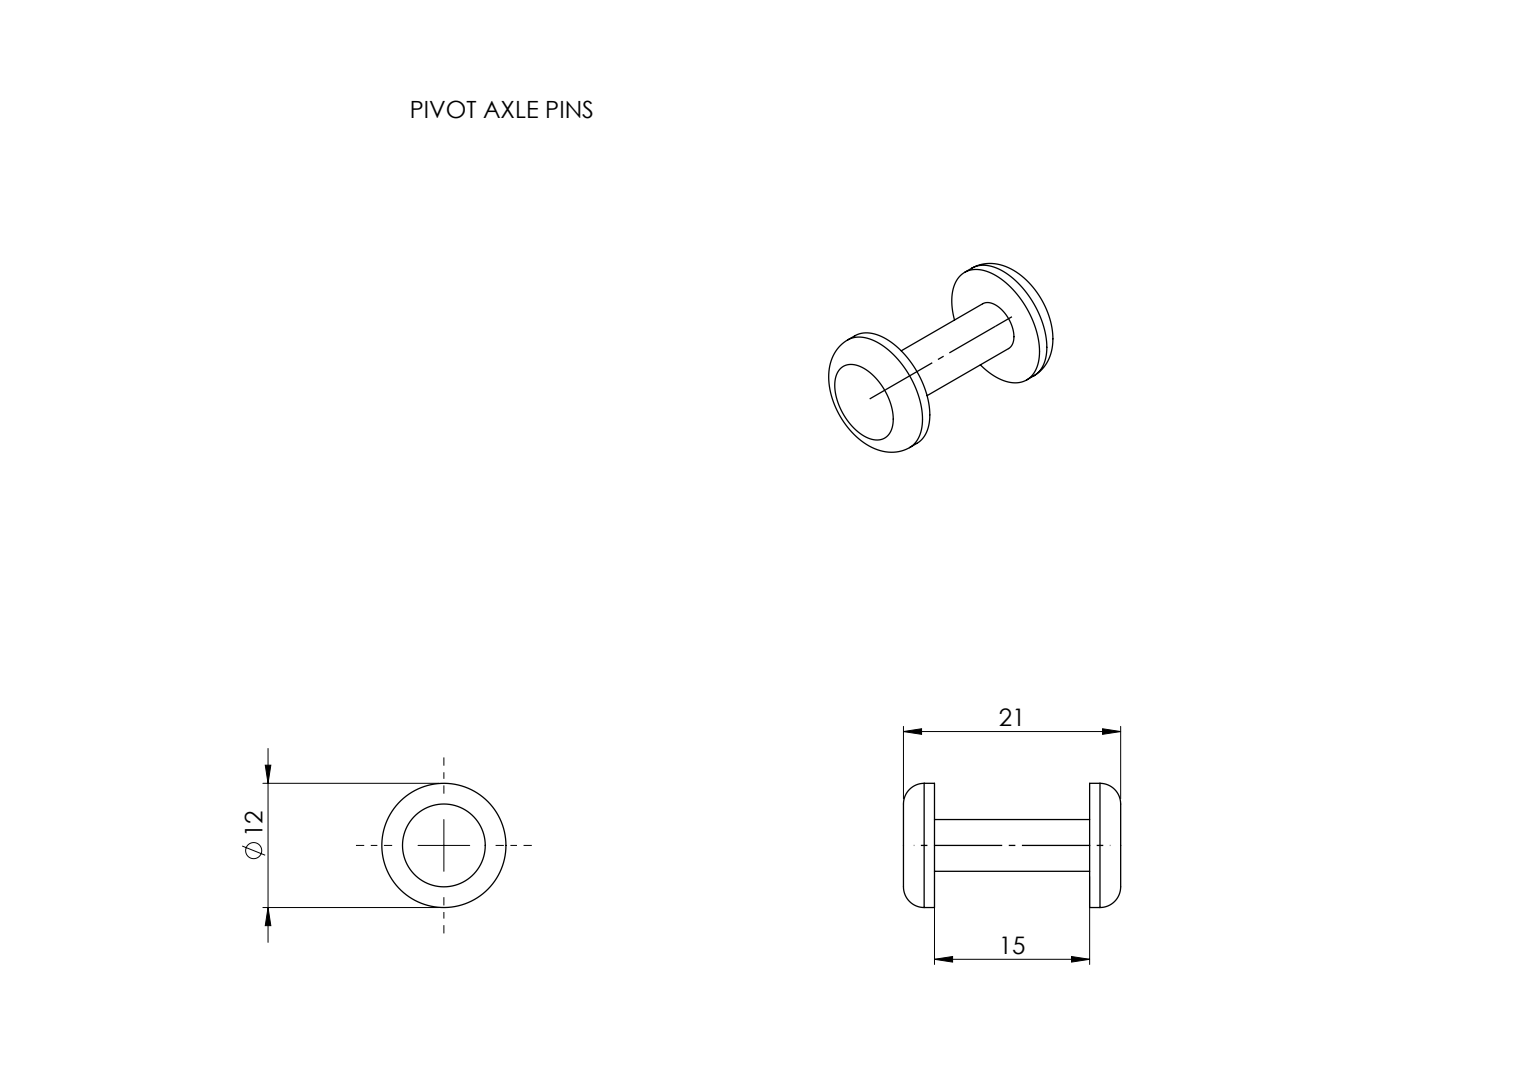
ISO-10303-21;
HEADER;
FILE_DESCRIPTION (('STEP AP214'),
    '1' );
FILE_NAME ('Pivot Axle Pins.step',
    '2026-10-08T14:03:35',
    ( '' ),
    ( '' ),
    'SwSTEP 2.0',
    'SolidWorks 2026',
    '' );
FILE_SCHEMA (( 'AUTOMOTIVE_DESIGN' ));
ENDSEC;

DATA;
#5=CIRCLE ( 'NONE', #8996, 5.999999999999998224 ) ;
#23=AXIS2_PLACEMENT_3D ( 'NONE', #10959, #4438, #5501 ) ;
#42=VERTEX_POINT ( 'NONE', #3602 ) ;
#77=FACE_BOUND ( 'NONE', #7085, .T. ) ;
#131=VERTEX_POINT ( 'NONE', #11545 ) ;
#137=AXIS2_PLACEMENT_3D ( 'NONE', #11805, #13167, #2478 ) ;
#178=DIRECTION ( 'NONE',  ( 1.000000000000000000, 0.000000000000000000, 0.000000000000000000 ) ) ;
#205=PLANE ( 'NONE',  #6332 ) ;
#210=ORIENTED_EDGE ( 'NONE', *, *, #10551, .T. ) ;
#257=DIRECTION ( 'NONE',  ( -0.000000000000000000, -0.000000000000000000, 1.000000000000000000 ) ) ;
#382=DIRECTION ( 'NONE',  ( 1.000000000000000000, 0.000000000000000000, 0.000000000000000000 ) ) ;
#411=FILL_AREA_STYLE_COLOUR ( '', #8311 ) ;
#418=ORIENTED_EDGE ( 'NONE', *, *, #4130, .F. ) ;
#427=EDGE_LOOP ( 'NONE', ( #12636, #418, #9896, #533 ) ) ;
#447=PLANE ( 'NONE',  #3696 ) ;
#454=AXIS2_PLACEMENT_3D ( 'NONE', #3228, #2248, #4282 ) ;
#492=PRODUCT_CONTEXT ( 'NONE', #10764, 'mechanical' ) ;
#533=ORIENTED_EDGE ( 'NONE', *, *, #2253, .T. ) ;
#560=EDGE_CURVE ( 'NONE', #8899, #4393, #6700, .T. ) ;
#567=CARTESIAN_POINT ( 'NONE',  ( -35.00000000000000000, -4.286263797015736496E-15, -7.500000000000000000 ) ) ;
#579=CARTESIAN_POINT ( 'NONE',  ( -41.00000000000000000, -4.286263797015736496E-15, 7.500000000000000000 ) ) ;
#591=SURFACE_STYLE_USAGE ( .BOTH. , #5908 ) ;
#768=VERTEX_POINT ( 'NONE', #9967 ) ;
#794=DIRECTION ( 'NONE',  ( 0.000000000000000000, 0.000000000000000000, 1.000000000000000000 ) ) ;
#835=CIRCLE ( 'NONE', #11129, 5.999999999999998224 ) ;
#888=CARTESIAN_POINT ( 'NONE',  ( -41.00000000000000000, -4.286263797015736496E-15, -10.49999999999999822 ) ) ;
#918=CYLINDRICAL_SURFACE ( 'NONE', #6361, 2.500000000000002220 ) ;
#963=LINE ( 'NONE', #2075, #5370 ) ;
#965=DIRECTION ( 'NONE',  ( -0.000000000000000000, -0.000000000000000000, -1.000000000000000000 ) ) ;
#1032=DIRECTION ( 'NONE',  ( -0.000000000000000000, -0.000000000000000000, -1.000000000000000000 ) ) ;
#1033=DIRECTION ( 'NONE',  ( -1.000000000000000000, 0.000000000000000000, 0.000000000000000000 ) ) ;
#1081=DIRECTION ( 'NONE',  ( -0.000000000000000000, -0.000000000000000000, 1.000000000000000000 ) ) ;
#1112=SURFACE_STYLE_USAGE ( .BOTH. , #4254 ) ;
#1158=ORIENTED_EDGE ( 'NONE', *, *, #4130, .T. ) ;
#1226=VERTEX_POINT ( 'NONE', #6896 ) ;
#1235=DIRECTION ( 'NONE',  ( 0.000000000000000000, 0.000000000000000000, -1.000000000000000000 ) ) ;
#1341=CARTESIAN_POINT ( 'NONE',  ( -39.00000000000000000, -4.776122516674677878E-15, -8.499999999999998224 ) ) ;
#1345=CARTESIAN_POINT ( 'NONE',  ( -35.00000000000000000, -4.286263797015736496E-15, -7.500000000000000000 ) ) ;
#1409=CARTESIAN_POINT ( 'NONE',  ( 0.000000000000000000, 0.000000000000000000, 0.000000000000000000 ) ) ;
#1434=CIRCLE ( 'NONE', #6806, 3.999999999999996447 ) ;
#1443=VECTOR ( 'NONE', #13173, 1000.000000000000000 ) ;
#1461=STYLED_ITEM ( 'NONE', ( #12222 ), #5559 ) ;
#1462=EDGE_LOOP ( 'NONE', ( #2845, #13234, #8779, #12885 ) ) ;
#1505=CARTESIAN_POINT ( 'NONE',  ( -35.00000000000000000, -4.286263797015736496E-15, 7.500000000000000000 ) ) ;
#1524=UNCERTAINTY_MEASURE_WITH_UNIT (LENGTH_MEASURE( 1.000000000000000082E-05 ), #2490, 'distance_accuracy_value', 'NONE');
#1595=STYLED_ITEM ( 'NONE', ( #6768 ), #7994 ) ;
#1604=ORIENTED_EDGE ( 'NONE', *, *, #8953, .F. ) ;
#1623=SHAPE_REPRESENTATION_RELATIONSHIP ( 'NONE' , 'NONE' ,  #3787, #5559 ) ;
#1647=CYLINDRICAL_SURFACE ( 'NONE', #7272, 5.999999999999998224 ) ;
#1667=CARTESIAN_POINT ( 'NONE',  ( -35.00000000000000000, -4.286263797015736496E-15, 10.49999999999999822 ) ) ;
#1691=AXIS2_PLACEMENT_3D ( 'NONE', #9348, #794, #9415 ) ;
#1746=CARTESIAN_POINT ( 'NONE',  ( -37.50000000000000711, -4.286263797015736496E-15, 7.500000000000000000 ) ) ;
#1782=CARTESIAN_POINT ( 'NONE',  ( -29.00000000000000355, -3.551475717527324818E-15, 8.499999999999998224 ) ) ;
#1783=DIRECTION ( 'NONE',  ( 0.000000000000000000, 0.000000000000000000, 1.000000000000000000 ) ) ;
#1851=CYLINDRICAL_SURFACE ( 'NONE', #13242, 5.999999999999998224 ) ;
#1939=DIRECTION ( 'NONE',  ( -0.000000000000000000, -0.000000000000000000, 1.000000000000000000 ) ) ;
#1990=VECTOR ( 'NONE', #3207, 1000.000000000000000 ) ;
#2036=CARTESIAN_POINT ( 'NONE',  ( -35.00000000000000000, -4.286263797015736496E-15, 7.500000000000000000 ) ) ;
#2075=CARTESIAN_POINT ( 'NONE',  ( -41.00000000000000000, -4.286263797015736496E-15, 10.49999999999999822 ) ) ;
#2089=LINE ( 'NONE', #5313, #1990 ) ;
#2155=CARTESIAN_POINT ( 'NONE',  ( -35.00000000000000000, -4.286263797015736496E-15, 10.49999999999999822 ) ) ;
#2225=AXIS2_PLACEMENT_3D ( 'NONE', #9848, #257, #4510 ) ;
#2247=EDGE_CURVE ( 'NONE', #4900, #4459, #5, .T. ) ;
#2248=DIRECTION ( 'NONE',  ( -0.000000000000000000, -0.000000000000000000, 1.000000000000000000 ) ) ;
#2253=EDGE_CURVE ( 'NONE', #12007, #13310, #11863, .T. ) ;
#2278=CARTESIAN_POINT ( 'NONE',  ( -35.00000000000000000, -4.286263797015736496E-15, -8.499999999999998224 ) ) ;
#2353=AXIS2_PLACEMENT_3D ( 'NONE', #10131, #5844, #11094 ) ;
#2414=TOROIDAL_SURFACE ( 'NONE', #9155, 3.999999999999998224, 2.000000000000000000 ) ;
#2478=DIRECTION ( 'NONE',  ( 1.000000000000000000, 0.000000000000000000, 0.000000000000000000 ) ) ;
#2490=( LENGTH_UNIT ( ) NAMED_UNIT ( * ) SI_UNIT ( .MILLI., .METRE. ) );
#2497=EDGE_CURVE ( 'NONE', #42, #4459, #963, .T. ) ;
#2580=CIRCLE ( 'NONE', #137, 3.999999999999996447 ) ;
#2658=ORIENTED_EDGE ( 'NONE', *, *, #11315, .T. ) ;
#2672=EDGE_CURVE ( 'NONE', #13647, #8899, #5165, .T. ) ;
#2673=EDGE_CURVE ( 'NONE', #8113, #42, #9191, .T. ) ;
#2756=VECTOR ( 'NONE', #8329, 1000.000000000000000 ) ;
#2766=EDGE_LOOP ( 'NONE', ( #12928, #8220 ) ) ;
#2810=ORIENTED_EDGE ( 'NONE', *, *, #3408, .F. ) ;
#2845=ORIENTED_EDGE ( 'NONE', *, *, #6497, .F. ) ;
#2885=FILL_AREA_STYLE ('',( #4706 ) ) ;
#2895=CIRCLE ( 'NONE', #3105, 2.500000000000002220 ) ;
#2897=EDGE_LOOP ( 'NONE', ( #1158, #7841 ) ) ;
#2955=CARTESIAN_POINT ( 'NONE',  ( -35.00000000000000000, -4.286263797015736496E-15, 7.500000000000000000 ) ) ;
#2983=AXIS2_PLACEMENT_3D ( 'NONE', #3063, #965, #13827 ) ;
#3035=MECHANICAL_DESIGN_GEOMETRIC_PRESENTATION_REPRESENTATION('',(#1461),#6605);
#3063=CARTESIAN_POINT ( 'NONE',  ( -35.00000000000000000, -4.286263797015736496E-15, 8.499999999999998224 ) ) ;
#3105=AXIS2_PLACEMENT_3D ( 'NONE', #567, #7912, #6713 ) ;
#3157=ORIENTED_EDGE ( 'NONE', *, *, #8437, .T. ) ;
#3207=DIRECTION ( 'NONE',  ( -0.000000000000000000, -0.000000000000000000, -1.000000000000000000 ) ) ;
#3227=VECTOR ( 'NONE', #1939, 1000.000000000000000 ) ;
#3228=CARTESIAN_POINT ( 'NONE',  ( -35.00000000000000000, -4.286263797015736496E-15, -10.49999999999999822 ) ) ;
#3286=PLANE ( 'NONE',  #11612 ) ;
#3317=DIRECTION ( 'NONE',  ( -1.000000000000000000, 1.224646799147353454E-16, 0.000000000000000000 ) ) ;
#3345=TOROIDAL_SURFACE ( 'NONE', #6937, 3.999999999999998224, 2.000000000000000000 ) ;
#3364=MECHANICAL_DESIGN_GEOMETRIC_PRESENTATION_REPRESENTATION('',(#1595),#8521);
#3392=CARTESIAN_POINT ( 'NONE',  ( -31.00000000000000711, -4.286263797015736496E-15, 10.49999999999999822 ) ) ;
#3408=EDGE_CURVE ( 'NONE', #8113, #12059, #3837, .T. ) ;
#3482=DIRECTION ( 'NONE',  ( 0.000000000000000000, 0.000000000000000000, -1.000000000000000000 ) ) ;
#3502=DIRECTION ( 'NONE',  ( -1.000000000000000000, 0.000000000000000000, 0.000000000000000000 ) ) ;
#3505=DIRECTION ( 'NONE',  ( 1.000000000000000000, 1.224646799147353454E-16, 0.000000000000000000 ) ) ;
#3513=DIRECTION ( 'NONE',  ( 0.000000000000000000, 0.000000000000000000, 1.000000000000000000 ) ) ;
#3583=EDGE_LOOP ( 'NONE', ( #5772, #5608, #6832, #5918 ) ) ;
#3589=DIRECTION ( 'NONE',  ( 1.000000000000000000, 0.000000000000000000, 0.000000000000000000 ) ) ;
#3602=CARTESIAN_POINT ( 'NONE',  ( -41.00000000000000000, -4.286263797015736496E-15, 8.499999999999998224 ) ) ;
#3628=ADVANCED_FACE ( 'NONE', ( #9017, #13324 ), #7110, .F. ) ;
#3691=SHAPE_DEFINITION_REPRESENTATION ( #13049, #3787 ) ;
#3696=AXIS2_PLACEMENT_3D ( 'NONE', #12146, #6813, #11088 ) ;
#3750=DIRECTION ( 'NONE',  ( 0.000000000000000000, 0.000000000000000000, 1.000000000000000000 ) ) ;
#3787=SHAPE_REPRESENTATION ( 'Pivot Axle Pins', ( #8193 ), #13606 ) ;
#3837=CIRCLE ( 'NONE', #11670, 2.000000000000000000 ) ;
#3913=AXIS2_PLACEMENT_3D ( 'NONE', #5709, #13099, #3317 ) ;
#3937=( LENGTH_UNIT ( ) NAMED_UNIT ( * ) SI_UNIT ( .MILLI., .METRE. ) );
#3954=DIRECTION ( 'NONE',  ( -0.000000000000000000, -0.000000000000000000, -1.000000000000000000 ) ) ;
#3996=AXIS2_PLACEMENT_3D ( 'NONE', #2155, #4392, #9664 ) ;
#4130=EDGE_CURVE ( 'NONE', #4461, #8031, #12976, .T. ) ;
#4136=DIRECTION ( 'NONE',  ( 1.000000000000000000, 0.000000000000000000, 0.000000000000000000 ) ) ;
#4155=PRODUCT_DEFINITION_FORMATION_WITH_SPECIFIED_SOURCE ( 'ANY', '', #9019, .NOT_KNOWN. ) ;
#4254=SURFACE_SIDE_STYLE ('',( #4588 ) ) ;
#4282=DIRECTION ( 'NONE',  ( 1.000000000000000000, 0.000000000000000000, 0.000000000000000000 ) ) ;
#4383=ADVANCED_FACE ( 'NONE', ( #77, #8614 ), #3286, .F. ) ;
#4392=DIRECTION ( 'NONE',  ( -0.000000000000000000, -0.000000000000000000, -1.000000000000000000 ) ) ;
#4393=VERTEX_POINT ( 'NONE', #9811 ) ;
#4438=DIRECTION ( 'NONE',  ( -0.000000000000000000, -0.000000000000000000, -1.000000000000000000 ) ) ;
#4441=CARTESIAN_POINT ( 'NONE',  ( -37.50000000000000711, -4.286263797015736496E-15, -7.500000000000000000 ) ) ;
#4458=ADVANCED_FACE ( 'NONE', ( #10306 ), #2414, .T. ) ;
#4459=VERTEX_POINT ( 'NONE', #579 ) ;
#4461=VERTEX_POINT ( 'NONE', #1746 ) ;
#4510=DIRECTION ( 'NONE',  ( 1.000000000000000000, 0.000000000000000000, 0.000000000000000000 ) ) ;
#4588=SURFACE_STYLE_FILL_AREA ( #12758 ) ;
#4592=CIRCLE ( 'NONE', #2353, 5.999999999999998224 ) ;
#4689=AXIS2_PLACEMENT_3D ( 'NONE', #4801, #8938, #3513 ) ;
#4706=FILL_AREA_STYLE_COLOUR ( '', #10205 ) ;
#4761=DIRECTION ( 'NONE',  ( 1.000000000000000000, 0.000000000000000000, 0.000000000000000000 ) ) ;
#4801=CARTESIAN_POINT ( 'NONE',  ( -31.00000000000000711, -4.286263797015736496E-15, -8.499999999999998224 ) ) ;
#4806=CARTESIAN_POINT ( 'NONE',  ( -41.00000000000000000, -4.286263797015736496E-15, -8.499999999999998224 ) ) ;
#4823=EDGE_CURVE ( 'NONE', #1226, #768, #835, .T. ) ;
#4900=VERTEX_POINT ( 'NONE', #8326 ) ;
#4936=CIRCLE ( 'NONE', #8724, 3.999999999999996447 ) ;
#5071=ORIENTED_EDGE ( 'NONE', *, *, #2672, .F. ) ;
#5076=DIRECTION ( 'NONE',  ( -1.000000000000000000, 0.000000000000000000, 0.000000000000000000 ) ) ;
#5115=ORIENTED_EDGE ( 'NONE', *, *, #5924, .T. ) ;
#5126=FACE_OUTER_BOUND ( 'NONE', #5614, .T. ) ;
#5165=CIRCLE ( 'NONE', #10093, 5.999999999999998224 ) ;
#5175=CARTESIAN_POINT ( 'NONE',  ( -31.00000000000000711, -4.286263797015736496E-15, 8.499999999999998224 ) ) ;
#5191=DIRECTION ( 'NONE',  ( 0.000000000000000000, 0.000000000000000000, 1.000000000000000000 ) ) ;
#5252=ORIENTED_EDGE ( 'NONE', *, *, #13339, .F. ) ;
#5299=DIRECTION ( 'NONE',  ( -0.000000000000000000, -0.000000000000000000, 1.000000000000000000 ) ) ;
#5313=CARTESIAN_POINT ( 'NONE',  ( -29.00000000000000355, -3.551475717527324818E-15, 10.49999999999999822 ) ) ;
#5348=CLOSED_SHELL ( 'NONE', ( #7075, #11998, #12703, #8925, #11450, #10014, #13692, #5636, #3628, #12289, #4383, #7452, #10791, #4458 ) ) ;
#5366=ORIENTED_EDGE ( 'NONE', *, *, #4823, .T. ) ;
#5370=VECTOR ( 'NONE', #1032, 1000.000000000000000 ) ;
#5501=DIRECTION ( 'NONE',  ( 1.000000000000000000, 0.000000000000000000, 0.000000000000000000 ) ) ;
#5549=CARTESIAN_POINT ( 'NONE',  ( -35.00000000000000000, -4.286263797015736496E-15, 7.500000000000000000 ) ) ;
#5556=CARTESIAN_POINT ( 'NONE',  ( -37.50000000000000711, -4.286263797015736496E-15, 7.500000000000000000 ) ) ;
#5559=ADVANCED_BREP_SHAPE_REPRESENTATION ( '', ( #7994, #8193 ), #13606 ) ;
#5581=CIRCLE ( 'NONE', #2225, 5.999999999999998224 ) ;
#5607=VERTEX_POINT ( 'NONE', #13196 ) ;
#5608=ORIENTED_EDGE ( 'NONE', *, *, #2673, .F. ) ;
#5614=EDGE_LOOP ( 'NONE', ( #11627, #210, #7003, #2810 ) ) ;
#5636=ADVANCED_FACE ( 'NONE', ( #7547 ), #205, .T. ) ;
#5639=FACE_OUTER_BOUND ( 'NONE', #10808, .T. ) ;
#5709=CARTESIAN_POINT ( 'NONE',  ( -39.00000000000000000, -3.796405077356795904E-15, 8.499999999999998224 ) ) ;
#5761=FACE_OUTER_BOUND ( 'NONE', #12496, .T. ) ;
#5772=ORIENTED_EDGE ( 'NONE', *, *, #10551, .F. ) ;
#5785=DIRECTION ( 'NONE',  ( 0.000000000000000000, 0.000000000000000000, -1.000000000000000000 ) ) ;
#5800=AXIS2_PLACEMENT_3D ( 'NONE', #10517, #5191, #4136 ) ;
#5825=ORIENTED_EDGE ( 'NONE', *, *, #2497, .T. ) ;
#5842=EDGE_CURVE ( 'NONE', #8031, #13310, #7403, .T. ) ;
#5844=DIRECTION ( 'NONE',  ( 0.000000000000000000, 0.000000000000000000, -1.000000000000000000 ) ) ;
#5882=DIRECTION ( 'NONE',  ( 0.000000000000000000, 0.000000000000000000, 1.000000000000000000 ) ) ;
#5908=SURFACE_SIDE_STYLE ('',( #10249 ) ) ;
#5917=ORIENTED_EDGE ( 'NONE', *, *, #13339, .T. ) ;
#5918=ORIENTED_EDGE ( 'NONE', *, *, #10219, .F. ) ;
#5924=EDGE_CURVE ( 'NONE', #42, #8113, #8346, .T. ) ;
#5968=DIRECTION ( 'NONE',  ( 1.000000000000000000, 0.000000000000000000, 0.000000000000000000 ) ) ;
#6049=( NAMED_UNIT ( * ) SI_UNIT ( $, .STERADIAN. ) SOLID_ANGLE_UNIT ( ) );
#6069=DIRECTION ( 'NONE',  ( 0.000000000000000000, 0.000000000000000000, 1.000000000000000000 ) ) ;
#6091=CARTESIAN_POINT ( 'NONE',  ( -32.50000000000000000, -3.980102097228898626E-15, 7.500000000000000000 ) ) ;
#6131=AXIS2_PLACEMENT_3D ( 'NONE', #2036, #10587, #8480 ) ;
#6194=DIRECTION ( 'NONE',  ( -1.000000000000000000, 0.000000000000000000, 0.000000000000000000 ) ) ;
#6332=AXIS2_PLACEMENT_3D ( 'NONE', #12039, #11764, #7683 ) ;
#6354=CYLINDRICAL_SURFACE ( 'NONE', #12250, 5.999999999999998224 ) ;
#6359=ORIENTED_EDGE ( 'NONE', *, *, #2253, .F. ) ;
#6361=AXIS2_PLACEMENT_3D ( 'NONE', #2955, #7221, #11504 ) ;
#6494=CIRCLE ( 'NONE', #10947, 5.999999999999998224 ) ;
#6497=EDGE_CURVE ( 'NONE', #8031, #4461, #11934, .T. ) ;
#6589=ORIENTED_EDGE ( 'NONE', *, *, #11075, .T. ) ;
#6605=( GEOMETRIC_REPRESENTATION_CONTEXT ( 3 ) GLOBAL_UNCERTAINTY_ASSIGNED_CONTEXT ( ( #13351 ) ) GLOBAL_UNIT_ASSIGNED_CONTEXT ( ( #3937, #8082, #6049 ) ) REPRESENTATION_CONTEXT ( 'NONE', 'WORKASPACE' ) );
#6634=ORIENTED_EDGE ( 'NONE', *, *, #560, .T. ) ;
#6700=CIRCLE ( 'NONE', #4689, 2.000000000000000000 ) ;
#6713=DIRECTION ( 'NONE',  ( 1.000000000000000000, 0.000000000000000000, 0.000000000000000000 ) ) ;
#6723=CARTESIAN_POINT ( 'NONE',  ( -35.00000000000000000, -4.286263797015736496E-15, -7.500000000000000000 ) ) ;
#6754=DIRECTION ( 'NONE',  ( 0.000000000000000000, 0.000000000000000000, 1.000000000000000000 ) ) ;
#6768=PRESENTATION_STYLE_ASSIGNMENT (( #1112 ) ) ;
#6806=AXIS2_PLACEMENT_3D ( 'NONE', #1667, #5882, #10223 ) ;
#6813=DIRECTION ( 'NONE',  ( 0.000000000000000000, 0.000000000000000000, -1.000000000000000000 ) ) ;
#6832=ORIENTED_EDGE ( 'NONE', *, *, #3408, .T. ) ;
#6842=( NAMED_UNIT ( * ) PLANE_ANGLE_UNIT ( ) SI_UNIT ( $, .RADIAN. ) );
#6896=CARTESIAN_POINT ( 'NONE',  ( -41.00000000000000000, -4.286263797015736496E-15, -7.500000000000000000 ) ) ;
#6937=AXIS2_PLACEMENT_3D ( 'NONE', #10958, #9714, #10818 ) ;
#7003=ORIENTED_EDGE ( 'NONE', *, *, #7538, .F. ) ;
#7010=APPLICATION_CONTEXT ( 'automotive_design' ) ;
#7044=CIRCLE ( 'NONE', #3913, 2.000000000000001776 ) ;
#7075=ADVANCED_FACE ( 'NONE', ( #5639 ), #3345, .T. ) ;
#7085=EDGE_LOOP ( 'NONE', ( #6359, #1604 ) ) ;
#7110=PLANE ( 'NONE',  #8756 ) ;
#7140=EDGE_CURVE ( 'NONE', #768, #1226, #5581, .T. ) ;
#7151=EDGE_CURVE ( 'NONE', #4459, #4900, #6494, .T. ) ;
#7160=CARTESIAN_POINT ( 'NONE',  ( -35.00000000000000000, -4.286263797015736496E-15, 7.500000000000000000 ) ) ;
#7179=FACE_OUTER_BOUND ( 'NONE', #10615, .T. ) ;
#7221=DIRECTION ( 'NONE',  ( -0.000000000000000000, -0.000000000000000000, -1.000000000000000000 ) ) ;
#7272=AXIS2_PLACEMENT_3D ( 'NONE', #13601, #3954, #5076 ) ;
#7317=FACE_OUTER_BOUND ( 'NONE', #3583, .T. ) ;
#7403=LINE ( 'NONE', #6091, #2756 ) ;
#7452=ADVANCED_FACE ( 'NONE', ( #7179 ), #1851, .T. ) ;
#7485=CYLINDRICAL_SURFACE ( 'NONE', #3996, 5.999999999999998224 ) ;
#7538=EDGE_CURVE ( 'NONE', #12059, #131, #4936, .T. ) ;
#7547=FACE_OUTER_BOUND ( 'NONE', #13469, .T. ) ;
#7569=ORIENTED_EDGE ( 'NONE', *, *, #8901, .F. ) ;
#7683=DIRECTION ( 'NONE',  ( 1.000000000000000000, 0.000000000000000000, -0.000000000000000000 ) ) ;
#7790=ORIENTED_EDGE ( 'NONE', *, *, #7151, .T. ) ;
#7841=ORIENTED_EDGE ( 'NONE', *, *, #6497, .T. ) ;
#7912=DIRECTION ( 'NONE',  ( 0.000000000000000000, 0.000000000000000000, 1.000000000000000000 ) ) ;
#7962=DIRECTION ( 'NONE',  ( 1.000000000000000000, 0.000000000000000000, 0.000000000000000000 ) ) ;
#7994=MANIFOLD_SOLID_BREP ( 'Mirror3', #5348 ) ;
#7996=CARTESIAN_POINT ( 'NONE',  ( -35.00000000000000000, -4.286263797015736496E-15, -8.499999999999998224 ) ) ;
#8031=VERTEX_POINT ( 'NONE', #12458 ) ;
#8055=PRODUCT_DEFINITION ( 'UNKNOWN', '', #4155, #12338 ) ;
#8082=( NAMED_UNIT ( * ) PLANE_ANGLE_UNIT ( ) SI_UNIT ( $, .RADIAN. ) );
#8113=VERTEX_POINT ( 'NONE', #1782 ) ;
#8193=AXIS2_PLACEMENT_3D ( 'NONE', #1409, #10931, #382 ) ;
#8220=ORIENTED_EDGE ( 'NONE', *, *, #2247, .F. ) ;
#8291=AXIS2_PLACEMENT_3D ( 'NONE', #1345, #12158, #178 ) ;
#8311=COLOUR_RGB ( '', 0.40784314, 0.44705882, 0.49803922) ;
#8326=CARTESIAN_POINT ( 'NONE',  ( -29.00000000000000355, -3.551475717527324818E-15, 7.500000000000000000 ) ) ;
#8329=DIRECTION ( 'NONE',  ( -0.000000000000000000, -0.000000000000000000, -1.000000000000000000 ) ) ;
#8346=CIRCLE ( 'NONE', #2983, 5.999999999999998224 ) ;
#8437=EDGE_CURVE ( 'NONE', #13647, #5607, #13663, .T. ) ;
#8480=DIRECTION ( 'NONE',  ( 1.000000000000000000, 0.000000000000000000, 0.000000000000000000 ) ) ;
#8521=( GEOMETRIC_REPRESENTATION_CONTEXT ( 3 ) GLOBAL_UNCERTAINTY_ASSIGNED_CONTEXT ( ( #1524 ) ) GLOBAL_UNIT_ASSIGNED_CONTEXT ( ( #2490, #6842, #11694 ) ) REPRESENTATION_CONTEXT ( 'NONE', 'WORKASPACE' ) );
#8614=FACE_OUTER_BOUND ( 'NONE', #12533, .T. ) ;
#8650=ORIENTED_EDGE ( 'NONE', *, *, #8901, .T. ) ;
#8698=DIRECTION ( 'NONE',  ( -0.000000000000000000, -0.000000000000000000, 1.000000000000000000 ) ) ;
#8724=AXIS2_PLACEMENT_3D ( 'NONE', #8774, #12872, #13086 ) ;
#8756=AXIS2_PLACEMENT_3D ( 'NONE', #10270, #3750, #11384 ) ;
#8774=CARTESIAN_POINT ( 'NONE',  ( -35.00000000000000000, -4.286263797015736496E-15, 10.49999999999999822 ) ) ;
#8779=ORIENTED_EDGE ( 'NONE', *, *, #8953, .T. ) ;
#8899=VERTEX_POINT ( 'NONE', #11696 ) ;
#8901=EDGE_CURVE ( 'NONE', #8113, #4900, #2089, .T. ) ;
#8925=ADVANCED_FACE ( 'NONE', ( #12841 ), #7485, .T. ) ;
#8938=DIRECTION ( 'NONE',  ( -0.000000000000000000, 1.000000000000000000, 0.000000000000000000 ) ) ;
#8953=EDGE_CURVE ( 'NONE', #13310, #12007, #2895, .T. ) ;
#8996=AXIS2_PLACEMENT_3D ( 'NONE', #5549, #6754, #3589 ) ;
#9017=FACE_BOUND ( 'NONE', #2897, .T. ) ;
#9019=PRODUCT ( 'Pivot Axle Pins', 'Pivot Axle Pins', '', ( #492 ) ) ;
#9054=ORIENTED_EDGE ( 'NONE', *, *, #2247, .T. ) ;
#9155=AXIS2_PLACEMENT_3D ( 'NONE', #7996, #12205, #5968 ) ;
#9191=CIRCLE ( 'NONE', #23, 5.999999999999998224 ) ;
#9249=ORIENTED_EDGE ( 'NONE', *, *, #560, .F. ) ;
#9250=ORIENTED_EDGE ( 'NONE', *, *, #2497, .F. ) ;
#9264=ORIENTED_EDGE ( 'NONE', *, *, #7538, .T. ) ;
#9286=FACE_OUTER_BOUND ( 'NONE', #11650, .T. ) ;
#9346=DIRECTION ( 'NONE',  ( -0.000000000000000000, -0.000000000000000000, -1.000000000000000000 ) ) ;
#9348=CARTESIAN_POINT ( 'NONE',  ( -35.00000000000000000, -4.286263797015736496E-15, 8.499999999999998224 ) ) ;
#9415=DIRECTION ( 'NONE',  ( 1.000000000000000000, 0.000000000000000000, 0.000000000000000000 ) ) ;
#9430=CARTESIAN_POINT ( 'NONE',  ( -35.00000000000000000, -4.286263797015736496E-15, -10.49999999999999822 ) ) ;
#9508=CARTESIAN_POINT ( 'NONE',  ( -32.50000000000000000, -3.980102097228898626E-15, -7.500000000000000000 ) ) ;
#9565=CARTESIAN_POINT ( 'NONE',  ( -35.00000000000000000, -4.286263797015736496E-15, 8.499999999999998224 ) ) ;
#9599=EDGE_LOOP ( 'NONE', ( #10727, #11247, #10354, #5252 ) ) ;
#9664=DIRECTION ( 'NONE',  ( -1.000000000000000000, 0.000000000000000000, 0.000000000000000000 ) ) ;
#9714=DIRECTION ( 'NONE',  ( 0.000000000000000000, 0.000000000000000000, -1.000000000000000000 ) ) ;
#9718=EDGE_CURVE ( 'NONE', #4393, #5607, #10294, .T. ) ;
#9758=LINE ( 'NONE', #12069, #10840 ) ;
#9811=CARTESIAN_POINT ( 'NONE',  ( -31.00000000000000711, -4.286263797015736496E-15, -10.49999999999999822 ) ) ;
#9848=CARTESIAN_POINT ( 'NONE',  ( -35.00000000000000000, -4.286263797015736496E-15, -7.500000000000000000 ) ) ;
#9896=ORIENTED_EDGE ( 'NONE', *, *, #10630, .T. ) ;
#9967=CARTESIAN_POINT ( 'NONE',  ( -29.00000000000000355, -5.021051876504148963E-15, -7.500000000000000000 ) ) ;
#10014=ADVANCED_FACE ( 'NONE', ( #13648 ), #918, .T. ) ;
#10039=( NAMED_UNIT ( * ) SI_UNIT ( $, .STERADIAN. ) SOLID_ANGLE_UNIT ( ) );
#10093=AXIS2_PLACEMENT_3D ( 'NONE', #2278, #1235, #12023 ) ;
#10131=CARTESIAN_POINT ( 'NONE',  ( -35.00000000000000000, -4.286263797015736496E-15, -8.499999999999998224 ) ) ;
#10163=ORIENTED_EDGE ( 'NONE', *, *, #9718, .T. ) ;
#10169=AXIS2_PLACEMENT_3D ( 'NONE', #9565, #1783, #13677 ) ;
#10205=COLOUR_RGB ( '', 0.40784314, 0.44705882, 0.49803922) ;
#10219=EDGE_CURVE ( 'NONE', #131, #12059, #1434, .T. ) ;
#10223=DIRECTION ( 'NONE',  ( 1.000000000000000000, 0.000000000000000000, 0.000000000000000000 ) ) ;
#10249=SURFACE_STYLE_FILL_AREA ( #2885 ) ;
#10270=CARTESIAN_POINT ( 'NONE',  ( -35.00000000000000000, -4.286263797015736496E-15, 7.500000000000000000 ) ) ;
#10294=CIRCLE ( 'NONE', #454, 3.999999999999996447 ) ;
#10306=FACE_OUTER_BOUND ( 'NONE', #12846, .T. ) ;
#10354=ORIENTED_EDGE ( 'NONE', *, *, #4823, .F. ) ;
#10390=ORIENTED_EDGE ( 'NONE', *, *, #10219, .T. ) ;
#10433=TOROIDAL_SURFACE ( 'NONE', #1691, 3.999999999999998224, 2.000000000000000000 ) ;
#10517=CARTESIAN_POINT ( 'NONE',  ( -35.00000000000000000, -4.286263797015736496E-15, 7.500000000000000000 ) ) ;
#10551=EDGE_CURVE ( 'NONE', #42, #131, #7044, .T. ) ;
#10587=DIRECTION ( 'NONE',  ( 0.000000000000000000, 0.000000000000000000, 1.000000000000000000 ) ) ;
#10615=EDGE_LOOP ( 'NONE', ( #11365, #5071, #5917, #11248 ) ) ;
#10625=CARTESIAN_POINT ( 'NONE',  ( -35.00000000000000000, -4.286263797015736496E-15, -10.49999999999999822 ) ) ;
#10630=EDGE_CURVE ( 'NONE', #4461, #12007, #13023, .T. ) ;
#10727=ORIENTED_EDGE ( 'NONE', *, *, #11315, .F. ) ;
#10764=APPLICATION_CONTEXT ( 'automotive_design' ) ;
#10778=DIRECTION ( 'NONE',  ( 1.000000000000000000, 0.000000000000000000, 0.000000000000000000 ) ) ;
#10784=EDGE_CURVE ( 'NONE', #8899, #768, #9758, .T. ) ;
#10791=ADVANCED_FACE ( 'NONE', ( #5761 ), #447, .T. ) ;
#10808=EDGE_LOOP ( 'NONE', ( #2658, #3157, #6589, #9249 ) ) ;
#10818=DIRECTION ( 'NONE',  ( 1.000000000000000000, 0.000000000000000000, 0.000000000000000000 ) ) ;
#10840=VECTOR ( 'NONE', #8698, 1000.000000000000000 ) ;
#10931=DIRECTION ( 'NONE',  ( 0.000000000000000000, 0.000000000000000000, 1.000000000000000000 ) ) ;
#10947=AXIS2_PLACEMENT_3D ( 'NONE', #1505, #6069, #7962 ) ;
#10958=CARTESIAN_POINT ( 'NONE',  ( -35.00000000000000000, -4.286263797015736496E-15, -8.499999999999998224 ) ) ;
#10959=CARTESIAN_POINT ( 'NONE',  ( -35.00000000000000000, -4.286263797015736496E-15, 8.499999999999998224 ) ) ;
#11075=EDGE_CURVE ( 'NONE', #5607, #4393, #2580, .T. ) ;
#11088=DIRECTION ( 'NONE',  ( 1.000000000000000000, 0.000000000000000000, 0.000000000000000000 ) ) ;
#11094=DIRECTION ( 'NONE',  ( 1.000000000000000000, 0.000000000000000000, 0.000000000000000000 ) ) ;
#11129=AXIS2_PLACEMENT_3D ( 'NONE', #12117, #12261, #4761 ) ;
#11164=( NAMED_UNIT ( * ) PLANE_ANGLE_UNIT ( ) SI_UNIT ( $, .RADIAN. ) );
#11195=ORIENTED_EDGE ( 'NONE', *, *, #9718, .F. ) ;
#11247=ORIENTED_EDGE ( 'NONE', *, *, #10784, .T. ) ;
#11248=ORIENTED_EDGE ( 'NONE', *, *, #7140, .F. ) ;
#11289=FACE_OUTER_BOUND ( 'NONE', #9599, .T. ) ;
#11315=EDGE_CURVE ( 'NONE', #8899, #13647, #4592, .T. ) ;
#11360=ORIENTED_EDGE ( 'NONE', *, *, #2672, .T. ) ;
#11365=ORIENTED_EDGE ( 'NONE', *, *, #10784, .F. ) ;
#11384=DIRECTION ( 'NONE',  ( 1.000000000000000000, 0.000000000000000000, -0.000000000000000000 ) ) ;
#11445=FACE_OUTER_BOUND ( 'NONE', #1462, .T. ) ;
#11450=ADVANCED_FACE ( 'NONE', ( #11445 ), #13728, .T. ) ;
#11504=DIRECTION ( 'NONE',  ( -1.000000000000000000, 0.000000000000000000, 0.000000000000000000 ) ) ;
#11545=CARTESIAN_POINT ( 'NONE',  ( -39.00000000000000000, -3.673940397442060756E-15, 10.49999999999999822 ) ) ;
#11612=AXIS2_PLACEMENT_3D ( 'NONE', #6723, #3482, #10778 ) ;
#11627=ORIENTED_EDGE ( 'NONE', *, *, #5924, .F. ) ;
#11650=EDGE_LOOP ( 'NONE', ( #7569, #12217, #5825, #7790 ) ) ;
#11670=AXIS2_PLACEMENT_3D ( 'NONE', #5175, #13176, #5785 ) ;
#11694=( NAMED_UNIT ( * ) SI_UNIT ( $, .STERADIAN. ) SOLID_ANGLE_UNIT ( ) );
#11696=CARTESIAN_POINT ( 'NONE',  ( -29.00000000000000355, -5.021051876504148963E-15, -8.499999999999998224 ) ) ;
#11764=DIRECTION ( 'NONE',  ( 0.000000000000000000, 0.000000000000000000, 1.000000000000000000 ) ) ;
#11805=CARTESIAN_POINT ( 'NONE',  ( -35.00000000000000000, -4.286263797015736496E-15, -10.49999999999999822 ) ) ;
#11863=CIRCLE ( 'NONE', #8291, 2.500000000000002220 ) ;
#11934=CIRCLE ( 'NONE', #6131, 2.500000000000002220 ) ;
#11961=ORIENTED_EDGE ( 'NONE', *, *, #8437, .F. ) ;
#11998=ADVANCED_FACE ( 'NONE', ( #11289 ), #6354, .T. ) ;
#12007=VERTEX_POINT ( 'NONE', #4441 ) ;
#12023=DIRECTION ( 'NONE',  ( 1.000000000000000000, 0.000000000000000000, 0.000000000000000000 ) ) ;
#12039=CARTESIAN_POINT ( 'NONE',  ( -35.00000000000000000, -4.286263797015736496E-15, 10.49999999999999822 ) ) ;
#12049=AXIS2_PLACEMENT_3D ( 'NONE', #1341, #13155, #3505 ) ;
#12057=ORIENTED_EDGE ( 'NONE', *, *, #7140, .T. ) ;
#12059=VERTEX_POINT ( 'NONE', #3392 ) ;
#12069=CARTESIAN_POINT ( 'NONE',  ( -29.00000000000000355, -5.021051876504148963E-15, -10.49999999999999822 ) ) ;
#12117=CARTESIAN_POINT ( 'NONE',  ( -35.00000000000000000, -4.286263797015736496E-15, -7.500000000000000000 ) ) ;
#12146=CARTESIAN_POINT ( 'NONE',  ( -35.00000000000000000, -4.286263797015736496E-15, -10.49999999999999822 ) ) ;
#12158=DIRECTION ( 'NONE',  ( 0.000000000000000000, 0.000000000000000000, 1.000000000000000000 ) ) ;
#12205=DIRECTION ( 'NONE',  ( 0.000000000000000000, 0.000000000000000000, -1.000000000000000000 ) ) ;
#12217=ORIENTED_EDGE ( 'NONE', *, *, #2673, .T. ) ;
#12222=PRESENTATION_STYLE_ASSIGNMENT (( #591 ) ) ;
#12250=AXIS2_PLACEMENT_3D ( 'NONE', #10625, #5299, #1033 ) ;
#12261=DIRECTION ( 'NONE',  ( -0.000000000000000000, -0.000000000000000000, 1.000000000000000000 ) ) ;
#12289=ADVANCED_FACE ( 'NONE', ( #7317 ), #13786, .T. ) ;
#12338=PRODUCT_DEFINITION_CONTEXT ( 'detailed design', #7010, 'design' ) ;
#12427=( LENGTH_UNIT ( ) NAMED_UNIT ( * ) SI_UNIT ( .MILLI., .METRE. ) );
#12458=CARTESIAN_POINT ( 'NONE',  ( -32.50000000000000000, -3.980102097228898626E-15, 7.500000000000000000 ) ) ;
#12496=EDGE_LOOP ( 'NONE', ( #11195, #13121 ) ) ;
#12533=EDGE_LOOP ( 'NONE', ( #5366, #12057 ) ) ;
#12636=ORIENTED_EDGE ( 'NONE', *, *, #5842, .F. ) ;
#12703=ADVANCED_FACE ( 'NONE', ( #5126 ), #10433, .T. ) ;
#12758=FILL_AREA_STYLE ('',( #411 ) ) ;
#12765=EDGE_LOOP ( 'NONE', ( #5115, #8650, #9054, #9250 ) ) ;
#12841=FACE_OUTER_BOUND ( 'NONE', #12765, .T. ) ;
#12846=EDGE_LOOP ( 'NONE', ( #11961, #11360, #6634, #10163 ) ) ;
#12872=DIRECTION ( 'NONE',  ( 0.000000000000000000, 0.000000000000000000, 1.000000000000000000 ) ) ;
#12885=ORIENTED_EDGE ( 'NONE', *, *, #10630, .F. ) ;
#12928=ORIENTED_EDGE ( 'NONE', *, *, #7151, .F. ) ;
#12976=CIRCLE ( 'NONE', #5800, 2.500000000000002220 ) ;
#13023=LINE ( 'NONE', #5556, #1443 ) ;
#13046=UNCERTAINTY_MEASURE_WITH_UNIT (LENGTH_MEASURE( 1.000000000000000082E-05 ), #12427, 'distance_accuracy_value', 'NONE');
#13049=PRODUCT_DEFINITION_SHAPE ( 'NONE', 'NONE',  #8055 ) ;
#13086=DIRECTION ( 'NONE',  ( 1.000000000000000000, 0.000000000000000000, 0.000000000000000000 ) ) ;
#13099=DIRECTION ( 'NONE',  ( 1.224646799147353207E-16, 1.000000000000000000, -0.000000000000000000 ) ) ;
#13121=ORIENTED_EDGE ( 'NONE', *, *, #11075, .F. ) ;
#13135=AXIS2_PLACEMENT_3D ( 'NONE', #7160, #9346, #6194 ) ;
#13155=DIRECTION ( 'NONE',  ( 1.224646799147353207E-16, -1.000000000000000000, 0.000000000000000000 ) ) ;
#13167=DIRECTION ( 'NONE',  ( -0.000000000000000000, -0.000000000000000000, 1.000000000000000000 ) ) ;
#13173=DIRECTION ( 'NONE',  ( -0.000000000000000000, -0.000000000000000000, -1.000000000000000000 ) ) ;
#13176=DIRECTION ( 'NONE',  ( 0.000000000000000000, -1.000000000000000000, 0.000000000000000000 ) ) ;
#13196=CARTESIAN_POINT ( 'NONE',  ( -39.00000000000000000, -4.898587196589413026E-15, -10.49999999999999822 ) ) ;
#13234=ORIENTED_EDGE ( 'NONE', *, *, #5842, .T. ) ;
#13242=AXIS2_PLACEMENT_3D ( 'NONE', #9430, #1081, #3502 ) ;
#13310=VERTEX_POINT ( 'NONE', #9508 ) ;
#13324=FACE_OUTER_BOUND ( 'NONE', #2766, .T. ) ;
#13339=EDGE_CURVE ( 'NONE', #13647, #1226, #13819, .T. ) ;
#13351=UNCERTAINTY_MEASURE_WITH_UNIT (LENGTH_MEASURE( 1.000000000000000082E-05 ), #3937, 'distance_accuracy_value', 'NONE');
#13469=EDGE_LOOP ( 'NONE', ( #9264, #10390 ) ) ;
#13601=CARTESIAN_POINT ( 'NONE',  ( -35.00000000000000000, -4.286263797015736496E-15, 10.49999999999999822 ) ) ;
#13606=( GEOMETRIC_REPRESENTATION_CONTEXT ( 3 ) GLOBAL_UNCERTAINTY_ASSIGNED_CONTEXT ( ( #13046 ) ) GLOBAL_UNIT_ASSIGNED_CONTEXT ( ( #12427, #11164, #10039 ) ) REPRESENTATION_CONTEXT ( 'NONE', 'WORKASPACE' ) );
#13647=VERTEX_POINT ( 'NONE', #4806 ) ;
#13648=FACE_OUTER_BOUND ( 'NONE', #427, .T. ) ;
#13663=CIRCLE ( 'NONE', #12049, 2.000000000000001776 ) ;
#13677=DIRECTION ( 'NONE',  ( 1.000000000000000000, 0.000000000000000000, 0.000000000000000000 ) ) ;
#13692=ADVANCED_FACE ( 'NONE', ( #9286 ), #1647, .T. ) ;
#13728=CYLINDRICAL_SURFACE ( 'NONE', #13135, 2.500000000000002220 ) ;
#13786=TOROIDAL_SURFACE ( 'NONE', #10169, 3.999999999999998224, 2.000000000000000000 ) ;
#13819=LINE ( 'NONE', #888, #3227 ) ;
#13827=DIRECTION ( 'NONE',  ( 1.000000000000000000, 0.000000000000000000, 0.000000000000000000 ) ) ;
ENDSEC;
END-ISO-10303-21;
